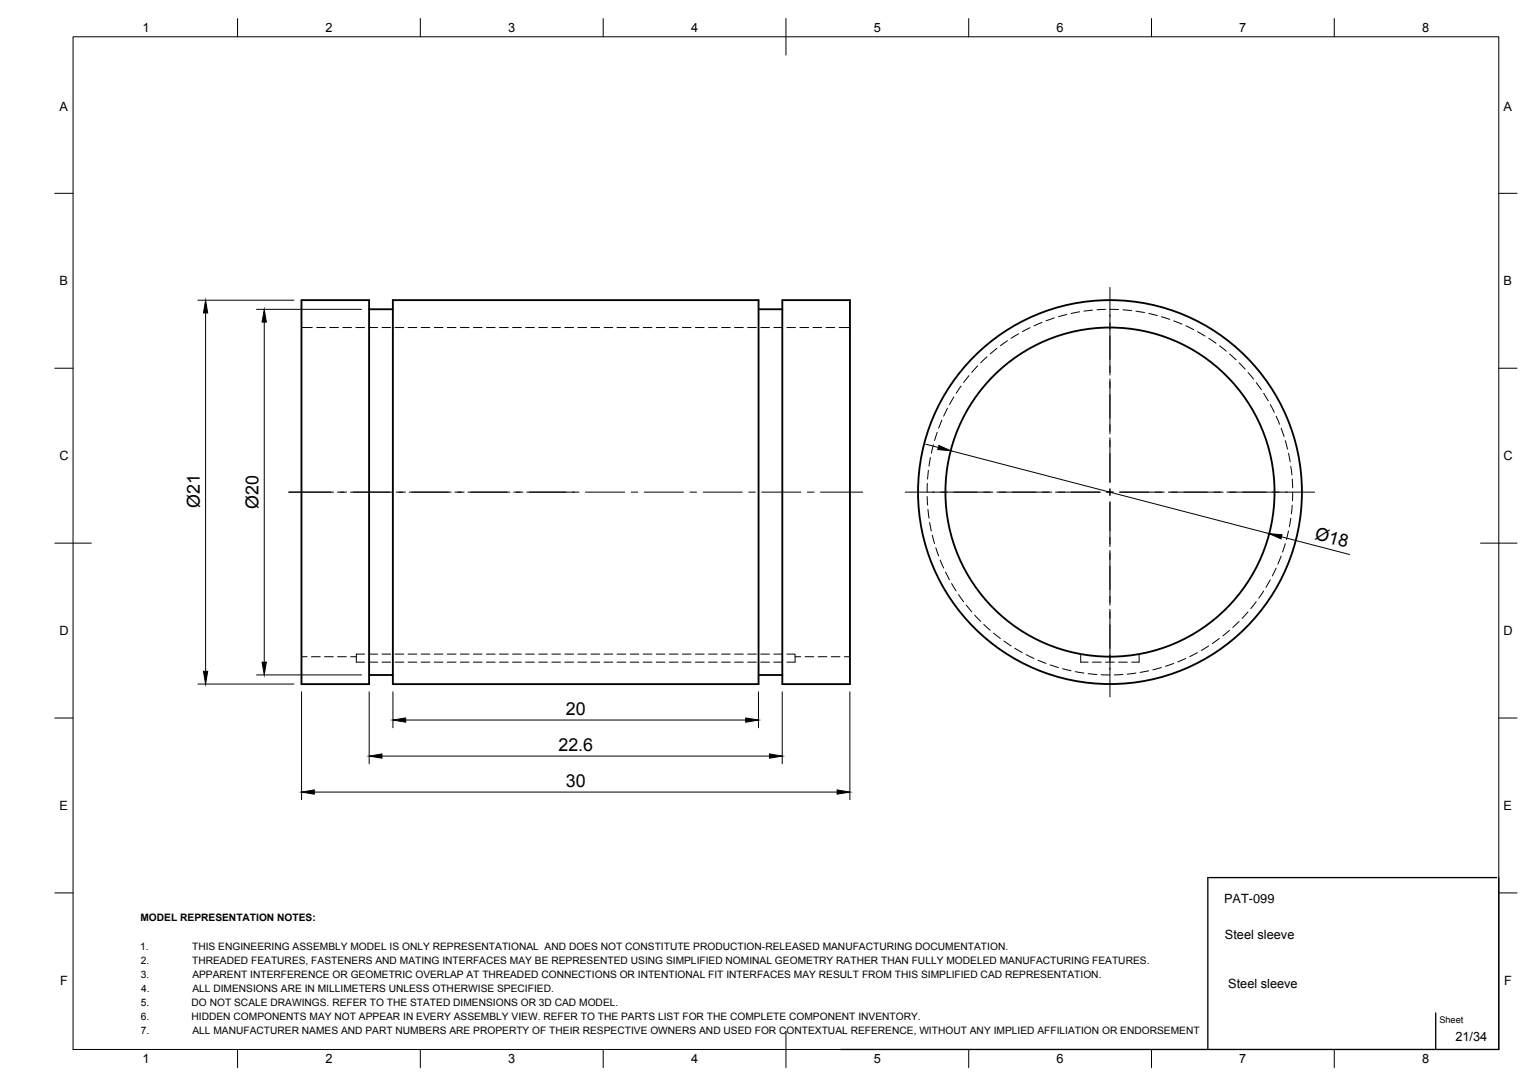
ISO-10303-21;
HEADER;
/* Generated by software containing ST-Developer
 * from STEP Tools, Inc. (www.steptools.com) 
 */

FILE_DESCRIPTION(
/* description */ ('PAT-099'),
/* implementation_level */ '2;1');

FILE_NAME(
/* name */ 'Steel sleeve.step',
/* time_stamp */ '2026-10-29T17:25:42-07:00',
/* author */ (''),
/* organization */ (''),
/* preprocessor_version */ 'ST-DEVELOPER v20.2',
/* originating_system */ 'Autodesk Translation Framework v15.17.0.0',
/* authorisation */ '');

FILE_SCHEMA (('AUTOMOTIVE_DESIGN { 1 0 10303 214 3 1 1 }'));
ENDSEC;

DATA;
#10=MECHANICAL_DESIGN_GEOMETRIC_PRESENTATION_REPRESENTATION('',(#344),#11035);
#294=SHAPE_REPRESENTATION_RELATIONSHIP('SRR','None',#11163,#319);
#319=ADVANCED_BREP_SHAPE_REPRESENTATION('',(#377),#11013);
#344=STYLED_ITEM('',(#11400),#377);
#377=MANIFOLD_SOLID_BREP('Body1',#4712);
#478=FACE_BOUND('',#1128,.T.);
#479=FACE_BOUND('',#1131,.T.);
#480=FACE_BOUND('',#1134,.T.);
#481=FACE_BOUND('',#1137,.T.);
#482=FACE_BOUND('',#1140,.T.);
#483=FACE_BOUND('',#1143,.T.);
#484=FACE_BOUND('',#1145,.T.);
#562=PLANE('',#5261);
#563=PLANE('',#5263);
#564=PLANE('',#5264);
#565=PLANE('',#5266);
#566=PLANE('',#5267);
#567=PLANE('',#5268);
#568=PLANE('',#5273);
#569=PLANE('',#5277);
#570=PLANE('',#5281);
#571=PLANE('',#5285);
#572=PLANE('',#5289);
#764=FACE_OUTER_BOUND('',#1122,.T.);
#765=FACE_OUTER_BOUND('',#1123,.T.);
#766=FACE_OUTER_BOUND('',#1124,.T.);
#767=FACE_OUTER_BOUND('',#1125,.T.);
#768=FACE_OUTER_BOUND('',#1126,.T.);
#769=FACE_OUTER_BOUND('',#1127,.T.);
#770=FACE_OUTER_BOUND('',#1129,.T.);
#771=FACE_OUTER_BOUND('',#1130,.T.);
#772=FACE_OUTER_BOUND('',#1132,.T.);
#773=FACE_OUTER_BOUND('',#1133,.T.);
#774=FACE_OUTER_BOUND('',#1135,.T.);
#775=FACE_OUTER_BOUND('',#1136,.T.);
#776=FACE_OUTER_BOUND('',#1138,.T.);
#777=FACE_OUTER_BOUND('',#1139,.T.);
#778=FACE_OUTER_BOUND('',#1141,.T.);
#779=FACE_OUTER_BOUND('',#1142,.T.);
#780=FACE_OUTER_BOUND('',#1144,.T.);
#1122=EDGE_LOOP('',(#3623,#3624,#3625,#3626));
#1123=EDGE_LOOP('',(#3627,#3628,#3629,#3630));
#1124=EDGE_LOOP('',(#3631,#3632,#3633,#3634));
#1125=EDGE_LOOP('',(#3635,#3636,#3637,#3638));
#1126=EDGE_LOOP('',(#3639,#3640,#3641,#3642));
#1127=EDGE_LOOP('',(#3643));
#1128=EDGE_LOOP('',(#3644));
#1129=EDGE_LOOP('',(#3645,#3646,#3647,#3648));
#1130=EDGE_LOOP('',(#3649));
#1131=EDGE_LOOP('',(#3650));
#1132=EDGE_LOOP('',(#3651,#3652,#3653,#3654));
#1133=EDGE_LOOP('',(#3655));
#1134=EDGE_LOOP('',(#3656));
#1135=EDGE_LOOP('',(#3657,#3658,#3659,#3660));
#1136=EDGE_LOOP('',(#3661));
#1137=EDGE_LOOP('',(#3662));
#1138=EDGE_LOOP('',(#3663,#3664,#3665,#3666));
#1139=EDGE_LOOP('',(#3667));
#1140=EDGE_LOOP('',(#3668));
#1141=EDGE_LOOP('',(#3669,#3670,#3671,#3672));
#1142=EDGE_LOOP('',(#3673));
#1143=EDGE_LOOP('',(#3674));
#1144=EDGE_LOOP('',(#3675,#3676,#3677,#3678));
#1145=EDGE_LOOP('',(#3679,#3680,#3681,#3682));
#1436=LINE('',#9751,#1688);
#1437=LINE('',#9753,#1689);
#1438=LINE('',#9754,#1690);
#1439=LINE('',#9757,#1691);
#1440=LINE('',#9759,#1692);
#1441=LINE('',#9760,#1693);
#1442=LINE('',#9765,#1694);
#1443=LINE('',#9766,#1695);
#1444=LINE('',#9768,#1696);
#1445=LINE('',#9769,#1697);
#1446=LINE('',#9779,#1698);
#1447=LINE('',#9786,#1699);
#1448=LINE('',#9793,#1700);
#1449=LINE('',#9800,#1701);
#1450=LINE('',#9807,#1702);
#1451=LINE('',#9812,#1703);
#1688=VECTOR('',#6255,1.);
#1689=VECTOR('',#6256,1.);
#1690=VECTOR('',#6257,1.);
#1691=VECTOR('',#6260,1.);
#1692=VECTOR('',#6261,1.);
#1693=VECTOR('',#6262,1.);
#1694=VECTOR('',#6267,1.);
#1695=VECTOR('',#6268,1.);
#1696=VECTOR('',#6271,1.);
#1697=VECTOR('',#6272,1.);
#1698=VECTOR('',#6285,1.05);
#1699=VECTOR('',#6294,1.);
#1700=VECTOR('',#6303,1.05);
#1701=VECTOR('',#6312,1.);
#1702=VECTOR('',#6321,1.05);
#1703=VECTOR('',#6328,0.9);
#1977=CIRCLE('',#5262,0.9);
#1978=CIRCLE('',#5265,0.9);
#1979=CIRCLE('',#5269,1.05);
#1980=CIRCLE('',#5270,0.9);
#1981=CIRCLE('',#5272,1.05);
#1982=CIRCLE('',#5274,1.);
#1983=CIRCLE('',#5276,1.);
#1984=CIRCLE('',#5278,1.05);
#1985=CIRCLE('',#5280,1.05);
#1986=CIRCLE('',#5282,1.);
#1987=CIRCLE('',#5284,1.);
#1988=CIRCLE('',#5286,1.05);
#1989=CIRCLE('',#5288,1.05);
#1990=CIRCLE('',#5290,0.9);
#2306=VERTEX_POINT('',#9747);
#2307=VERTEX_POINT('',#9748);
#2308=VERTEX_POINT('',#9750);
#2309=VERTEX_POINT('',#9752);
#2310=VERTEX_POINT('',#9756);
#2311=VERTEX_POINT('',#9758);
#2312=VERTEX_POINT('',#9762);
#2313=VERTEX_POINT('',#9764);
#2314=VERTEX_POINT('',#9772);
#2315=VERTEX_POINT('',#9774);
#2316=VERTEX_POINT('',#9777);
#2317=VERTEX_POINT('',#9781);
#2318=VERTEX_POINT('',#9784);
#2319=VERTEX_POINT('',#9788);
#2320=VERTEX_POINT('',#9791);
#2321=VERTEX_POINT('',#9795);
#2322=VERTEX_POINT('',#9798);
#2323=VERTEX_POINT('',#9802);
#2324=VERTEX_POINT('',#9805);
#2325=VERTEX_POINT('',#9809);
#2788=EDGE_CURVE('',#2306,#2307,#1977,.T.);
#2789=EDGE_CURVE('',#2308,#2306,#1436,.T.);
#2790=EDGE_CURVE('',#2309,#2308,#1437,.T.);
#2791=EDGE_CURVE('',#2307,#2309,#1438,.T.);
#2792=EDGE_CURVE('',#2307,#2310,#1439,.T.);
#2793=EDGE_CURVE('',#2311,#2309,#1440,.T.);
#2794=EDGE_CURVE('',#2311,#2310,#1441,.T.);
#2795=EDGE_CURVE('',#2310,#2312,#1978,.T.);
#2796=EDGE_CURVE('',#2313,#2311,#1442,.T.);
#2797=EDGE_CURVE('',#2312,#2313,#1443,.T.);
#2798=EDGE_CURVE('',#2312,#2306,#1444,.T.);
#2799=EDGE_CURVE('',#2313,#2308,#1445,.T.);
#2800=EDGE_CURVE('',#2314,#2314,#1979,.T.);
#2801=EDGE_CURVE('',#2315,#2315,#1980,.T.);
#2802=EDGE_CURVE('',#2316,#2316,#1981,.T.);
#2803=EDGE_CURVE('',#2316,#2314,#1446,.T.);
#2804=EDGE_CURVE('',#2317,#2317,#1982,.T.);
#2805=EDGE_CURVE('',#2318,#2318,#1983,.T.);
#2806=EDGE_CURVE('',#2318,#2317,#1447,.T.);
#2807=EDGE_CURVE('',#2319,#2319,#1984,.T.);
#2808=EDGE_CURVE('',#2320,#2320,#1985,.T.);
#2809=EDGE_CURVE('',#2320,#2319,#1448,.T.);
#2810=EDGE_CURVE('',#2321,#2321,#1986,.T.);
#2811=EDGE_CURVE('',#2322,#2322,#1987,.T.);
#2812=EDGE_CURVE('',#2322,#2321,#1449,.T.);
#2813=EDGE_CURVE('',#2323,#2323,#1988,.T.);
#2814=EDGE_CURVE('',#2324,#2324,#1989,.T.);
#2815=EDGE_CURVE('',#2324,#2323,#1450,.T.);
#2816=EDGE_CURVE('',#2325,#2325,#1990,.T.);
#2817=EDGE_CURVE('',#2325,#2315,#1451,.T.);
#3623=ORIENTED_EDGE('',*,*,#2788,.F.);
#3624=ORIENTED_EDGE('',*,*,#2789,.F.);
#3625=ORIENTED_EDGE('',*,*,#2790,.F.);
#3626=ORIENTED_EDGE('',*,*,#2791,.F.);
#3627=ORIENTED_EDGE('',*,*,#2792,.F.);
#3628=ORIENTED_EDGE('',*,*,#2791,.T.);
#3629=ORIENTED_EDGE('',*,*,#2793,.F.);
#3630=ORIENTED_EDGE('',*,*,#2794,.T.);
#3631=ORIENTED_EDGE('',*,*,#2795,.F.);
#3632=ORIENTED_EDGE('',*,*,#2794,.F.);
#3633=ORIENTED_EDGE('',*,*,#2796,.F.);
#3634=ORIENTED_EDGE('',*,*,#2797,.F.);
#3635=ORIENTED_EDGE('',*,*,#2798,.F.);
#3636=ORIENTED_EDGE('',*,*,#2797,.T.);
#3637=ORIENTED_EDGE('',*,*,#2799,.T.);
#3638=ORIENTED_EDGE('',*,*,#2789,.T.);
#3639=ORIENTED_EDGE('',*,*,#2799,.F.);
#3640=ORIENTED_EDGE('',*,*,#2796,.T.);
#3641=ORIENTED_EDGE('',*,*,#2793,.T.);
#3642=ORIENTED_EDGE('',*,*,#2790,.T.);
#3643=ORIENTED_EDGE('',*,*,#2800,.F.);
#3644=ORIENTED_EDGE('',*,*,#2801,.T.);
#3645=ORIENTED_EDGE('',*,*,#2802,.F.);
#3646=ORIENTED_EDGE('',*,*,#2803,.T.);
#3647=ORIENTED_EDGE('',*,*,#2800,.T.);
#3648=ORIENTED_EDGE('',*,*,#2803,.F.);
#3649=ORIENTED_EDGE('',*,*,#2802,.T.);
#3650=ORIENTED_EDGE('',*,*,#2804,.F.);
#3651=ORIENTED_EDGE('',*,*,#2805,.F.);
#3652=ORIENTED_EDGE('',*,*,#2806,.T.);
#3653=ORIENTED_EDGE('',*,*,#2804,.T.);
#3654=ORIENTED_EDGE('',*,*,#2806,.F.);
#3655=ORIENTED_EDGE('',*,*,#2807,.F.);
#3656=ORIENTED_EDGE('',*,*,#2805,.T.);
#3657=ORIENTED_EDGE('',*,*,#2808,.F.);
#3658=ORIENTED_EDGE('',*,*,#2809,.T.);
#3659=ORIENTED_EDGE('',*,*,#2807,.T.);
#3660=ORIENTED_EDGE('',*,*,#2809,.F.);
#3661=ORIENTED_EDGE('',*,*,#2808,.T.);
#3662=ORIENTED_EDGE('',*,*,#2810,.F.);
#3663=ORIENTED_EDGE('',*,*,#2811,.F.);
#3664=ORIENTED_EDGE('',*,*,#2812,.T.);
#3665=ORIENTED_EDGE('',*,*,#2810,.T.);
#3666=ORIENTED_EDGE('',*,*,#2812,.F.);
#3667=ORIENTED_EDGE('',*,*,#2813,.F.);
#3668=ORIENTED_EDGE('',*,*,#2811,.T.);
#3669=ORIENTED_EDGE('',*,*,#2814,.F.);
#3670=ORIENTED_EDGE('',*,*,#2815,.T.);
#3671=ORIENTED_EDGE('',*,*,#2813,.T.);
#3672=ORIENTED_EDGE('',*,*,#2815,.F.);
#3673=ORIENTED_EDGE('',*,*,#2814,.T.);
#3674=ORIENTED_EDGE('',*,*,#2816,.F.);
#3675=ORIENTED_EDGE('',*,*,#2816,.T.);
#3676=ORIENTED_EDGE('',*,*,#2817,.T.);
#3677=ORIENTED_EDGE('',*,*,#2801,.F.);
#3678=ORIENTED_EDGE('',*,*,#2817,.F.);
#3679=ORIENTED_EDGE('',*,*,#2795,.T.);
#3680=ORIENTED_EDGE('',*,*,#2798,.T.);
#3681=ORIENTED_EDGE('',*,*,#2788,.T.);
#3682=ORIENTED_EDGE('',*,*,#2792,.T.);
#4374=CYLINDRICAL_SURFACE('',#5271,1.05);
#4375=CYLINDRICAL_SURFACE('',#5275,1.);
#4376=CYLINDRICAL_SURFACE('',#5279,1.05);
#4377=CYLINDRICAL_SURFACE('',#5283,1.);
#4378=CYLINDRICAL_SURFACE('',#5287,1.05);
#4379=CYLINDRICAL_SURFACE('',#5291,0.9);
#4529=ADVANCED_FACE('',(#764),#562,.F.);
#4530=ADVANCED_FACE('',(#765),#563,.F.);
#4531=ADVANCED_FACE('',(#766),#564,.F.);
#4532=ADVANCED_FACE('',(#767),#565,.F.);
#4533=ADVANCED_FACE('',(#768),#566,.F.);
#4534=ADVANCED_FACE('',(#769,#478),#567,.T.);
#4535=ADVANCED_FACE('',(#770),#4374,.T.);
#4536=ADVANCED_FACE('',(#771,#479),#568,.T.);
#4537=ADVANCED_FACE('',(#772),#4375,.T.);
#4538=ADVANCED_FACE('',(#773,#480),#569,.T.);
#4539=ADVANCED_FACE('',(#774),#4376,.T.);
#4540=ADVANCED_FACE('',(#775,#481),#570,.T.);
#4541=ADVANCED_FACE('',(#776),#4377,.T.);
#4542=ADVANCED_FACE('',(#777,#482),#571,.T.);
#4543=ADVANCED_FACE('',(#778),#4378,.T.);
#4544=ADVANCED_FACE('',(#779,#483),#572,.T.);
#4545=ADVANCED_FACE('',(#780,#484),#4379,.F.);
#4712=CLOSED_SHELL('',(#4529,#4530,#4531,#4532,#4533,#4534,#4535,#4536,
#4537,#4538,#4539,#4540,#4541,#4542,#4543,#4544,#4545));
#5260=AXIS2_PLACEMENT_3D('',#9745,#6249,#6250);
#5261=AXIS2_PLACEMENT_3D('',#9746,#6251,#6252);
#5262=AXIS2_PLACEMENT_3D('',#9749,#6253,#6254);
#5263=AXIS2_PLACEMENT_3D('',#9755,#6258,#6259);
#5264=AXIS2_PLACEMENT_3D('',#9761,#6263,#6264);
#5265=AXIS2_PLACEMENT_3D('',#9763,#6265,#6266);
#5266=AXIS2_PLACEMENT_3D('',#9767,#6269,#6270);
#5267=AXIS2_PLACEMENT_3D('',#9770,#6273,#6274);
#5268=AXIS2_PLACEMENT_3D('',#9771,#6275,#6276);
#5269=AXIS2_PLACEMENT_3D('',#9773,#6277,#6278);
#5270=AXIS2_PLACEMENT_3D('',#9775,#6279,#6280);
#5271=AXIS2_PLACEMENT_3D('',#9776,#6281,#6282);
#5272=AXIS2_PLACEMENT_3D('',#9778,#6283,#6284);
#5273=AXIS2_PLACEMENT_3D('',#9780,#6286,#6287);
#5274=AXIS2_PLACEMENT_3D('',#9782,#6288,#6289);
#5275=AXIS2_PLACEMENT_3D('',#9783,#6290,#6291);
#5276=AXIS2_PLACEMENT_3D('',#9785,#6292,#6293);
#5277=AXIS2_PLACEMENT_3D('',#9787,#6295,#6296);
#5278=AXIS2_PLACEMENT_3D('',#9789,#6297,#6298);
#5279=AXIS2_PLACEMENT_3D('',#9790,#6299,#6300);
#5280=AXIS2_PLACEMENT_3D('',#9792,#6301,#6302);
#5281=AXIS2_PLACEMENT_3D('',#9794,#6304,#6305);
#5282=AXIS2_PLACEMENT_3D('',#9796,#6306,#6307);
#5283=AXIS2_PLACEMENT_3D('',#9797,#6308,#6309);
#5284=AXIS2_PLACEMENT_3D('',#9799,#6310,#6311);
#5285=AXIS2_PLACEMENT_3D('',#9801,#6313,#6314);
#5286=AXIS2_PLACEMENT_3D('',#9803,#6315,#6316);
#5287=AXIS2_PLACEMENT_3D('',#9804,#6317,#6318);
#5288=AXIS2_PLACEMENT_3D('',#9806,#6319,#6320);
#5289=AXIS2_PLACEMENT_3D('',#9808,#6322,#6323);
#5290=AXIS2_PLACEMENT_3D('',#9810,#6324,#6325);
#5291=AXIS2_PLACEMENT_3D('',#9811,#6326,#6327);
#6249=DIRECTION('axis',(0.,0.,1.));
#6250=DIRECTION('refdir',(1.,0.,0.));
#6251=DIRECTION('center_axis',(0.,1.,0.));
#6252=DIRECTION('ref_axis',(0.,0.,1.));
#6253=DIRECTION('center_axis',(0.,-1.,0.));
#6254=DIRECTION('ref_axis',(1.,0.,0.));
#6255=DIRECTION('',(-1.,0.,0.));
#6256=DIRECTION('',(0.,0.,-1.));
#6257=DIRECTION('',(1.,0.,0.));
#6258=DIRECTION('center_axis',(0.,0.,1.));
#6259=DIRECTION('ref_axis',(1.,0.,0.));
#6260=DIRECTION('',(0.,-1.,0.));
#6261=DIRECTION('',(0.,1.,0.));
#6262=DIRECTION('',(-1.,0.,0.));
#6263=DIRECTION('center_axis',(0.,-1.,0.));
#6264=DIRECTION('ref_axis',(0.,0.,-1.));
#6265=DIRECTION('center_axis',(0.,1.,0.));
#6266=DIRECTION('ref_axis',(1.,0.,0.));
#6267=DIRECTION('',(0.,0.,1.));
#6268=DIRECTION('',(1.,0.,0.));
#6269=DIRECTION('center_axis',(0.,0.,-1.));
#6270=DIRECTION('ref_axis',(-1.,0.,0.));
#6271=DIRECTION('',(0.,1.,0.));
#6272=DIRECTION('',(0.,1.,0.));
#6273=DIRECTION('center_axis',(1.,0.,0.));
#6274=DIRECTION('ref_axis',(0.,0.,-1.));
#6275=DIRECTION('center_axis',(0.,1.,0.));
#6276=DIRECTION('ref_axis',(0.,0.,1.));
#6277=DIRECTION('center_axis',(0.,-1.,0.));
#6278=DIRECTION('ref_axis',(1.,0.,0.));
#6279=DIRECTION('center_axis',(0.,-1.,0.));
#6280=DIRECTION('ref_axis',(1.,0.,0.));
#6281=DIRECTION('center_axis',(0.,-1.,0.));
#6282=DIRECTION('ref_axis',(1.,0.,0.));
#6283=DIRECTION('center_axis',(0.,-1.,0.));
#6284=DIRECTION('ref_axis',(1.,0.,0.));
#6285=DIRECTION('',(0.,1.,0.));
#6286=DIRECTION('center_axis',(0.,-1.,0.));
#6287=DIRECTION('ref_axis',(0.,0.,-1.));
#6288=DIRECTION('center_axis',(0.,-1.,0.));
#6289=DIRECTION('ref_axis',(1.,0.,0.));
#6290=DIRECTION('center_axis',(0.,-1.,0.));
#6291=DIRECTION('ref_axis',(1.,0.,0.));
#6292=DIRECTION('center_axis',(0.,-1.,0.));
#6293=DIRECTION('ref_axis',(1.,0.,0.));
#6294=DIRECTION('',(0.,1.,0.));
#6295=DIRECTION('center_axis',(0.,1.,0.));
#6296=DIRECTION('ref_axis',(0.,0.,1.));
#6297=DIRECTION('center_axis',(0.,-1.,0.));
#6298=DIRECTION('ref_axis',(1.,0.,0.));
#6299=DIRECTION('center_axis',(0.,-1.,0.));
#6300=DIRECTION('ref_axis',(1.,0.,0.));
#6301=DIRECTION('center_axis',(0.,-1.,0.));
#6302=DIRECTION('ref_axis',(1.,0.,0.));
#6303=DIRECTION('',(0.,1.,0.));
#6304=DIRECTION('center_axis',(0.,-1.,0.));
#6305=DIRECTION('ref_axis',(0.,0.,-1.));
#6306=DIRECTION('center_axis',(0.,-1.,0.));
#6307=DIRECTION('ref_axis',(1.,0.,0.));
#6308=DIRECTION('center_axis',(0.,-1.,0.));
#6309=DIRECTION('ref_axis',(1.,0.,0.));
#6310=DIRECTION('center_axis',(0.,-1.,0.));
#6311=DIRECTION('ref_axis',(1.,0.,0.));
#6312=DIRECTION('',(0.,1.,0.));
#6313=DIRECTION('center_axis',(0.,1.,0.));
#6314=DIRECTION('ref_axis',(0.,0.,1.));
#6315=DIRECTION('center_axis',(0.,-1.,0.));
#6316=DIRECTION('ref_axis',(1.,0.,0.));
#6317=DIRECTION('center_axis',(0.,-1.,0.));
#6318=DIRECTION('ref_axis',(1.,0.,0.));
#6319=DIRECTION('center_axis',(0.,-1.,0.));
#6320=DIRECTION('ref_axis',(1.,0.,0.));
#6321=DIRECTION('',(0.,1.,0.));
#6322=DIRECTION('center_axis',(0.,-1.,0.));
#6323=DIRECTION('ref_axis',(0.,0.,-1.));
#6324=DIRECTION('center_axis',(0.,-1.,0.));
#6325=DIRECTION('ref_axis',(1.,0.,0.));
#6326=DIRECTION('center_axis',(0.,-1.,0.));
#6327=DIRECTION('ref_axis',(1.,0.,0.));
#6328=DIRECTION('',(0.,1.,0.));
#9745=CARTESIAN_POINT('',(0.,0.,0.));
#9746=CARTESIAN_POINT('Origin',(0.75,1.2,0.));
#9747=CARTESIAN_POINT('',(0.885663593019381,1.2,-0.16));
#9748=CARTESIAN_POINT('',(0.885663593019381,1.2,0.16));
#9749=CARTESIAN_POINT('Origin',(0.,1.2,0.));
#9750=CARTESIAN_POINT('',(0.93,1.2,-0.16));
#9751=CARTESIAN_POINT('',(0.93,1.2,-0.16));
#9752=CARTESIAN_POINT('',(0.93,1.2,0.16));
#9753=CARTESIAN_POINT('',(0.93,1.2,0.16));
#9754=CARTESIAN_POINT('',(0.57,1.2,0.16));
#9755=CARTESIAN_POINT('Origin',(0.57,0.,0.16));
#9756=CARTESIAN_POINT('',(0.885663593019381,-1.2,0.16));
#9757=CARTESIAN_POINT('',(0.885663593019381,0.,0.16));
#9758=CARTESIAN_POINT('',(0.93,-1.2,0.16));
#9759=CARTESIAN_POINT('',(0.93,0.,0.16));
#9760=CARTESIAN_POINT('',(0.57,-1.2,0.16));
#9761=CARTESIAN_POINT('Origin',(0.75,-1.2,0.));
#9762=CARTESIAN_POINT('',(0.885663593019381,-1.2,-0.16));
#9763=CARTESIAN_POINT('Origin',(0.,-1.2,0.));
#9764=CARTESIAN_POINT('',(0.93,-1.2,-0.16));
#9765=CARTESIAN_POINT('',(0.93,-1.2,0.16));
#9766=CARTESIAN_POINT('',(0.93,-1.2,-0.16));
#9767=CARTESIAN_POINT('Origin',(0.93,0.,-0.16));
#9768=CARTESIAN_POINT('',(0.885663593019381,0.,-0.16));
#9769=CARTESIAN_POINT('',(0.93,0.,-0.16));
#9770=CARTESIAN_POINT('Origin',(0.93,0.,0.16));
#9771=CARTESIAN_POINT('Origin',(1.05,1.5,0.));
#9772=CARTESIAN_POINT('',(-1.05,1.5,-1.28587913910472E-16));
#9773=CARTESIAN_POINT('Origin',(0.,1.5,0.));
#9774=CARTESIAN_POINT('',(-0.9,1.5,-1.10218211923262E-16));
#9775=CARTESIAN_POINT('Origin',(0.,1.5,0.));
#9776=CARTESIAN_POINT('Origin',(0.,1.315,0.));
#9777=CARTESIAN_POINT('',(-1.05,1.13,-1.28587913910472E-16));
#9778=CARTESIAN_POINT('Origin',(0.,1.13,0.));
#9779=CARTESIAN_POINT('',(-1.05,1.315,-1.28587913910472E-16));
#9780=CARTESIAN_POINT('Origin',(1.,1.13,0.));
#9781=CARTESIAN_POINT('',(-1.,1.13,-1.22464679914735E-16));
#9782=CARTESIAN_POINT('Origin',(0.,1.13,0.));
#9783=CARTESIAN_POINT('Origin',(0.,1.065,0.));
#9784=CARTESIAN_POINT('',(-1.,1.,-1.22464679914735E-16));
#9785=CARTESIAN_POINT('Origin',(0.,1.,0.));
#9786=CARTESIAN_POINT('',(-1.,1.065,-1.22464679914735E-16));
#9787=CARTESIAN_POINT('Origin',(1.05,1.,0.));
#9788=CARTESIAN_POINT('',(-1.05,1.,-1.28587913910472E-16));
#9789=CARTESIAN_POINT('Origin',(0.,1.,0.));
#9790=CARTESIAN_POINT('Origin',(0.,0.,0.));
#9791=CARTESIAN_POINT('',(-1.05,-1.,-1.28587913910472E-16));
#9792=CARTESIAN_POINT('Origin',(0.,-1.,0.));
#9793=CARTESIAN_POINT('',(-1.05,0.,-1.28587913910472E-16));
#9794=CARTESIAN_POINT('Origin',(1.,-1.,0.));
#9795=CARTESIAN_POINT('',(-1.,-1.,-1.22464679914735E-16));
#9796=CARTESIAN_POINT('Origin',(0.,-1.,0.));
#9797=CARTESIAN_POINT('Origin',(0.,-1.065,0.));
#9798=CARTESIAN_POINT('',(-1.,-1.13,-1.22464679914735E-16));
#9799=CARTESIAN_POINT('Origin',(0.,-1.13,0.));
#9800=CARTESIAN_POINT('',(-1.,-1.065,-1.22464679914735E-16));
#9801=CARTESIAN_POINT('Origin',(1.05,-1.13,0.));
#9802=CARTESIAN_POINT('',(-1.05,-1.13,-1.28587913910472E-16));
#9803=CARTESIAN_POINT('Origin',(0.,-1.13,0.));
#9804=CARTESIAN_POINT('Origin',(0.,-1.315,0.));
#9805=CARTESIAN_POINT('',(-1.05,-1.5,-1.28587913910472E-16));
#9806=CARTESIAN_POINT('Origin',(0.,-1.5,0.));
#9807=CARTESIAN_POINT('',(-1.05,-1.315,-1.28587913910472E-16));
#9808=CARTESIAN_POINT('Origin',(0.9,-1.5,0.));
#9809=CARTESIAN_POINT('',(-0.9,-1.5,-1.10218211923262E-16));
#9810=CARTESIAN_POINT('Origin',(0.,-1.5,0.));
#9811=CARTESIAN_POINT('Origin',(0.,0.,0.));
#9812=CARTESIAN_POINT('',(-0.9,0.,-1.10218211923262E-16));
#10980=UNCERTAINTY_MEASURE_WITH_UNIT(LENGTH_MEASURE(0.001),#11036,
'DISTANCE_ACCURACY_VALUE',
'Maximum model space distance between geometric entities at asserted c
onnectivities');
#11002=UNCERTAINTY_MEASURE_WITH_UNIT(LENGTH_MEASURE(0.001),#11036,
'DISTANCE_ACCURACY_VALUE',
'Maximum model space distance between geometric entities at asserted c
onnectivities');
#11013=(
GEOMETRIC_REPRESENTATION_CONTEXT(3)
GLOBAL_UNCERTAINTY_ASSIGNED_CONTEXT((#10980))
GLOBAL_UNIT_ASSIGNED_CONTEXT((#11036,#11038,#11039))
REPRESENTATION_CONTEXT('','3D')
);
#11035=(
GEOMETRIC_REPRESENTATION_CONTEXT(3)
GLOBAL_UNCERTAINTY_ASSIGNED_CONTEXT((#11002))
GLOBAL_UNIT_ASSIGNED_CONTEXT((#11036,#11038,#11039))
REPRESENTATION_CONTEXT('','3D')
);
#11036=(
LENGTH_UNIT()
NAMED_UNIT(*)
SI_UNIT(.CENTI.,.METRE.)
);
#11038=(
NAMED_UNIT(*)
PLANE_ANGLE_UNIT()
SI_UNIT($,.RADIAN.)
);
#11039=(
NAMED_UNIT(*)
SI_UNIT($,.STERADIAN.)
SOLID_ANGLE_UNIT()
);
#11050=SHAPE_DEFINITION_REPRESENTATION(#11082,#11163);
#11082=PRODUCT_DEFINITION_SHAPE('',$,#11196);
#11163=SHAPE_REPRESENTATION('',(#5260),#11013);
#11185=PRODUCT_DEFINITION_CONTEXT('part definition',#11283,'design');
#11196=PRODUCT_DEFINITION('Steel sleeve','Steel sleeve',#11228,#11185);
#11228=PRODUCT_DEFINITION_FORMATION('',$,#11295);
#11283=APPLICATION_CONTEXT(
'Core Data for Automotive Mechanical Design Process');
#11284=PRODUCT_CONTEXT('part definition',#11283,'mechanical');
#11295=PRODUCT('Steel sleeve','Steel sleeve','Steel sleeve',(#11284));
#11394=COLOUR_RGB('Off White',0.89,0.88,0.83);
#11395=FILL_AREA_STYLE_COLOUR('',#11394);
#11396=FILL_AREA_STYLE('',(#11395));
#11397=SURFACE_STYLE_FILL_AREA(#11396);
#11398=SURFACE_SIDE_STYLE('',(#11397));
#11399=SURFACE_STYLE_USAGE(.BOTH.,#11398);
#11400=PRESENTATION_STYLE_ASSIGNMENT((#11399));
ENDSEC;
END-ISO-10303-21;
